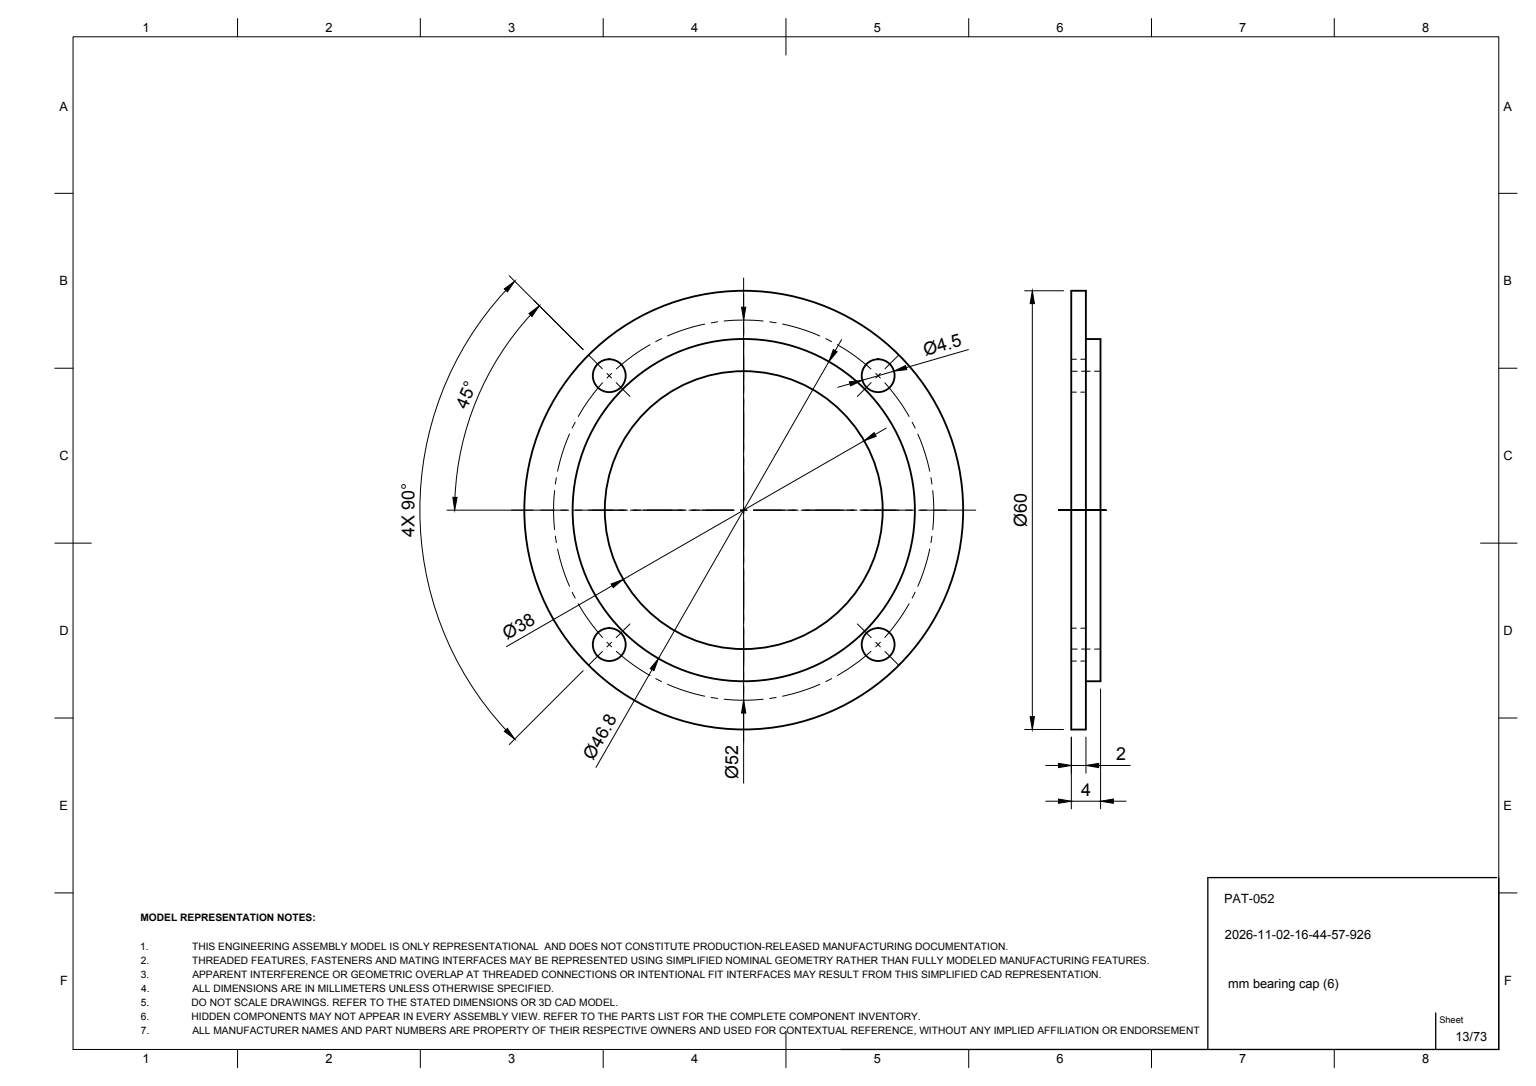
ISO-10303-21;
HEADER;
/* Generated by software containing ST-Developer
 * from STEP Tools, Inc. (www.steptools.com) 
 */

FILE_DESCRIPTION(
/* description */ ('Hand-crank gear train demonstrator'),
/* implementation_level */ '2;1');

FILE_NAME(
/* name */ 'mm bearing cap (6).step',
/* time_stamp */ '2026-10-28T03:22:13-07:00',
/* author */ (''),
/* organization */ (''),
/* preprocessor_version */ 'ST-DEVELOPER v20.2',
/* originating_system */ 'Autodesk Translation Framework v15.17.0.0',
/* authorisation */ '');

FILE_SCHEMA (('AUTOMOTIVE_DESIGN { 1 0 10303 214 3 1 1 }'));
ENDSEC;

DATA;
#10=MECHANICAL_DESIGN_GEOMETRIC_PRESENTATION_REPRESENTATION('',(#1198),#62758);
#1070=SHAPE_REPRESENTATION_RELATIONSHIP('SRR','None',#63042,#1134);
#1134=ADVANCED_BREP_SHAPE_REPRESENTATION('',(#1276),#62696);
#1198=STYLED_ITEM('',(#63462),#1276);
#1276=MANIFOLD_SOLID_BREP('Body1',#16379);
#1465=FACE_BOUND('',#3306,.T.);
#1466=FACE_BOUND('',#3310,.T.);
#1467=FACE_BOUND('',#3311,.T.);
#1468=FACE_BOUND('',#3312,.T.);
#1469=FACE_BOUND('',#3313,.T.);
#1470=FACE_BOUND('',#3314,.T.);
#1471=FACE_BOUND('',#3316,.T.);
#1472=FACE_BOUND('',#3317,.T.);
#1473=FACE_BOUND('',#3318,.T.);
#1474=FACE_BOUND('',#3319,.T.);
#1475=FACE_BOUND('',#3320,.T.);
#1676=PLANE('',#17450);
#1677=PLANE('',#17457);
#1678=PLANE('',#17458);
#2241=FACE_OUTER_BOUND('',#3300,.T.);
#2242=FACE_OUTER_BOUND('',#3301,.T.);
#2243=FACE_OUTER_BOUND('',#3302,.T.);
#2244=FACE_OUTER_BOUND('',#3303,.T.);
#2245=FACE_OUTER_BOUND('',#3304,.T.);
#2246=FACE_OUTER_BOUND('',#3305,.T.);
#2247=FACE_OUTER_BOUND('',#3307,.T.);
#2248=FACE_OUTER_BOUND('',#3308,.T.);
#2249=FACE_OUTER_BOUND('',#3309,.T.);
#2250=FACE_OUTER_BOUND('',#3315,.T.);
#3300=EDGE_LOOP('',(#11375,#11376,#11377,#11378));
#3301=EDGE_LOOP('',(#11379,#11380,#11381,#11382));
#3302=EDGE_LOOP('',(#11383,#11384,#11385,#11386));
#3303=EDGE_LOOP('',(#11387,#11388,#11389,#11390));
#3304=EDGE_LOOP('',(#11391,#11392,#11393,#11394));
#3305=EDGE_LOOP('',(#11395));
#3306=EDGE_LOOP('',(#11396));
#3307=EDGE_LOOP('',(#11397,#11398,#11399,#11400));
#3308=EDGE_LOOP('',(#11401,#11402,#11403,#11404));
#3309=EDGE_LOOP('',(#11405));
#3310=EDGE_LOOP('',(#11406));
#3311=EDGE_LOOP('',(#11407));
#3312=EDGE_LOOP('',(#11408));
#3313=EDGE_LOOP('',(#11409));
#3314=EDGE_LOOP('',(#11410));
#3315=EDGE_LOOP('',(#11411));
#3316=EDGE_LOOP('',(#11412));
#3317=EDGE_LOOP('',(#11413));
#3318=EDGE_LOOP('',(#11414));
#3319=EDGE_LOOP('',(#11415));
#3320=EDGE_LOOP('',(#11416));
#4409=LINE('',#23892,#5541);
#4410=LINE('',#23898,#5542);
#4411=LINE('',#23904,#5543);
#4412=LINE('',#23910,#5544);
#4413=LINE('',#23916,#5545);
#4414=LINE('',#23923,#5546);
#4415=LINE('',#23929,#5547);
#5541=VECTOR('',#19512,0.225000000000001);
#5542=VECTOR('',#19519,0.225000000000001);
#5543=VECTOR('',#19526,0.225000000000001);
#5544=VECTOR('',#19533,0.225000000000001);
#5545=VECTOR('',#19540,2.34);
#5546=VECTOR('',#19549,1.9);
#5547=VECTOR('',#19556,3.);
#6697=CIRCLE('',#17436,0.225000000000001);
#6698=CIRCLE('',#17437,0.225000000000001);
#6699=CIRCLE('',#17439,0.225000000000001);
#6700=CIRCLE('',#17440,0.225000000000001);
#6701=CIRCLE('',#17442,0.225000000000001);
#6702=CIRCLE('',#17443,0.225000000000001);
#6703=CIRCLE('',#17445,0.225000000000001);
#6704=CIRCLE('',#17446,0.225000000000001);
#6705=CIRCLE('',#17448,2.34);
#6706=CIRCLE('',#17449,2.34);
#6707=CIRCLE('',#17451,1.9);
#6708=CIRCLE('',#17453,1.9);
#6709=CIRCLE('',#17455,3.);
#6710=CIRCLE('',#17456,3.);
#7391=VERTEX_POINT('',#23889);
#7392=VERTEX_POINT('',#23891);
#7393=VERTEX_POINT('',#23895);
#7394=VERTEX_POINT('',#23897);
#7395=VERTEX_POINT('',#23901);
#7396=VERTEX_POINT('',#23903);
#7397=VERTEX_POINT('',#23907);
#7398=VERTEX_POINT('',#23909);
#7399=VERTEX_POINT('',#23913);
#7400=VERTEX_POINT('',#23915);
#7401=VERTEX_POINT('',#23919);
#7402=VERTEX_POINT('',#23922);
#7403=VERTEX_POINT('',#23926);
#7404=VERTEX_POINT('',#23928);
#8939=EDGE_CURVE('',#7391,#7391,#6697,.T.);
#8940=EDGE_CURVE('',#7391,#7392,#4409,.T.);
#8941=EDGE_CURVE('',#7392,#7392,#6698,.T.);
#8942=EDGE_CURVE('',#7393,#7393,#6699,.T.);
#8943=EDGE_CURVE('',#7393,#7394,#4410,.T.);
#8944=EDGE_CURVE('',#7394,#7394,#6700,.T.);
#8945=EDGE_CURVE('',#7395,#7395,#6701,.T.);
#8946=EDGE_CURVE('',#7395,#7396,#4411,.T.);
#8947=EDGE_CURVE('',#7396,#7396,#6702,.T.);
#8948=EDGE_CURVE('',#7397,#7397,#6703,.T.);
#8949=EDGE_CURVE('',#7397,#7398,#4412,.T.);
#8950=EDGE_CURVE('',#7398,#7398,#6704,.T.);
#8951=EDGE_CURVE('',#7399,#7399,#6705,.T.);
#8952=EDGE_CURVE('',#7399,#7400,#4413,.T.);
#8953=EDGE_CURVE('',#7400,#7400,#6706,.T.);
#8954=EDGE_CURVE('',#7401,#7401,#6707,.T.);
#8955=EDGE_CURVE('',#7401,#7402,#4414,.T.);
#8956=EDGE_CURVE('',#7402,#7402,#6708,.T.);
#8957=EDGE_CURVE('',#7403,#7403,#6709,.T.);
#8958=EDGE_CURVE('',#7403,#7404,#4415,.T.);
#8959=EDGE_CURVE('',#7404,#7404,#6710,.T.);
#11375=ORIENTED_EDGE('',*,*,#8939,.F.);
#11376=ORIENTED_EDGE('',*,*,#8940,.T.);
#11377=ORIENTED_EDGE('',*,*,#8941,.F.);
#11378=ORIENTED_EDGE('',*,*,#8940,.F.);
#11379=ORIENTED_EDGE('',*,*,#8942,.F.);
#11380=ORIENTED_EDGE('',*,*,#8943,.T.);
#11381=ORIENTED_EDGE('',*,*,#8944,.F.);
#11382=ORIENTED_EDGE('',*,*,#8943,.F.);
#11383=ORIENTED_EDGE('',*,*,#8945,.F.);
#11384=ORIENTED_EDGE('',*,*,#8946,.T.);
#11385=ORIENTED_EDGE('',*,*,#8947,.F.);
#11386=ORIENTED_EDGE('',*,*,#8946,.F.);
#11387=ORIENTED_EDGE('',*,*,#8948,.F.);
#11388=ORIENTED_EDGE('',*,*,#8949,.T.);
#11389=ORIENTED_EDGE('',*,*,#8950,.F.);
#11390=ORIENTED_EDGE('',*,*,#8949,.F.);
#11391=ORIENTED_EDGE('',*,*,#8951,.F.);
#11392=ORIENTED_EDGE('',*,*,#8952,.T.);
#11393=ORIENTED_EDGE('',*,*,#8953,.F.);
#11394=ORIENTED_EDGE('',*,*,#8952,.F.);
#11395=ORIENTED_EDGE('',*,*,#8951,.T.);
#11396=ORIENTED_EDGE('',*,*,#8954,.T.);
#11397=ORIENTED_EDGE('',*,*,#8954,.F.);
#11398=ORIENTED_EDGE('',*,*,#8955,.T.);
#11399=ORIENTED_EDGE('',*,*,#8956,.T.);
#11400=ORIENTED_EDGE('',*,*,#8955,.F.);
#11401=ORIENTED_EDGE('',*,*,#8957,.F.);
#11402=ORIENTED_EDGE('',*,*,#8958,.T.);
#11403=ORIENTED_EDGE('',*,*,#8959,.T.);
#11404=ORIENTED_EDGE('',*,*,#8958,.F.);
#11405=ORIENTED_EDGE('',*,*,#8957,.T.);
#11406=ORIENTED_EDGE('',*,*,#8953,.T.);
#11407=ORIENTED_EDGE('',*,*,#8950,.T.);
#11408=ORIENTED_EDGE('',*,*,#8947,.T.);
#11409=ORIENTED_EDGE('',*,*,#8944,.T.);
#11410=ORIENTED_EDGE('',*,*,#8941,.T.);
#11411=ORIENTED_EDGE('',*,*,#8959,.F.);
#11412=ORIENTED_EDGE('',*,*,#8956,.F.);
#11413=ORIENTED_EDGE('',*,*,#8948,.T.);
#11414=ORIENTED_EDGE('',*,*,#8945,.T.);
#11415=ORIENTED_EDGE('',*,*,#8942,.T.);
#11416=ORIENTED_EDGE('',*,*,#8939,.T.);
#15239=CYLINDRICAL_SURFACE('',#17435,0.225000000000001);
#15240=CYLINDRICAL_SURFACE('',#17438,0.225000000000001);
#15241=CYLINDRICAL_SURFACE('',#17441,0.225000000000001);
#15242=CYLINDRICAL_SURFACE('',#17444,0.225000000000001);
#15243=CYLINDRICAL_SURFACE('',#17447,2.34);
#15244=CYLINDRICAL_SURFACE('',#17452,1.9);
#15245=CYLINDRICAL_SURFACE('',#17454,3.);
#15551=ADVANCED_FACE('',(#2241),#15239,.F.);
#15552=ADVANCED_FACE('',(#2242),#15240,.F.);
#15553=ADVANCED_FACE('',(#2243),#15241,.F.);
#15554=ADVANCED_FACE('',(#2244),#15242,.F.);
#15555=ADVANCED_FACE('',(#2245),#15243,.T.);
#15556=ADVANCED_FACE('',(#2246,#1465),#1676,.T.);
#15557=ADVANCED_FACE('',(#2247),#15244,.F.);
#15558=ADVANCED_FACE('',(#2248),#15245,.T.);
#15559=ADVANCED_FACE('',(#2249,#1466,#1467,#1468,#1469,#1470),#1677,.T.);
#15560=ADVANCED_FACE('',(#2250,#1471,#1472,#1473,#1474,#1475),#1678,.F.);
#16379=CLOSED_SHELL('',(#15551,#15552,#15553,#15554,#15555,#15556,#15557,
#15558,#15559,#15560));
#17434=AXIS2_PLACEMENT_3D('',#23887,#19506,#19507);
#17435=AXIS2_PLACEMENT_3D('',#23888,#19508,#19509);
#17436=AXIS2_PLACEMENT_3D('',#23890,#19510,#19511);
#17437=AXIS2_PLACEMENT_3D('',#23893,#19513,#19514);
#17438=AXIS2_PLACEMENT_3D('',#23894,#19515,#19516);
#17439=AXIS2_PLACEMENT_3D('',#23896,#19517,#19518);
#17440=AXIS2_PLACEMENT_3D('',#23899,#19520,#19521);
#17441=AXIS2_PLACEMENT_3D('',#23900,#19522,#19523);
#17442=AXIS2_PLACEMENT_3D('',#23902,#19524,#19525);
#17443=AXIS2_PLACEMENT_3D('',#23905,#19527,#19528);
#17444=AXIS2_PLACEMENT_3D('',#23906,#19529,#19530);
#17445=AXIS2_PLACEMENT_3D('',#23908,#19531,#19532);
#17446=AXIS2_PLACEMENT_3D('',#23911,#19534,#19535);
#17447=AXIS2_PLACEMENT_3D('',#23912,#19536,#19537);
#17448=AXIS2_PLACEMENT_3D('',#23914,#19538,#19539);
#17449=AXIS2_PLACEMENT_3D('',#23917,#19541,#19542);
#17450=AXIS2_PLACEMENT_3D('',#23918,#19543,#19544);
#17451=AXIS2_PLACEMENT_3D('',#23920,#19545,#19546);
#17452=AXIS2_PLACEMENT_3D('',#23921,#19547,#19548);
#17453=AXIS2_PLACEMENT_3D('',#23924,#19550,#19551);
#17454=AXIS2_PLACEMENT_3D('',#23925,#19552,#19553);
#17455=AXIS2_PLACEMENT_3D('',#23927,#19554,#19555);
#17456=AXIS2_PLACEMENT_3D('',#23930,#19557,#19558);
#17457=AXIS2_PLACEMENT_3D('',#23931,#19559,#19560);
#17458=AXIS2_PLACEMENT_3D('',#23932,#19561,#19562);
#19506=DIRECTION('axis',(0.,0.,1.));
#19507=DIRECTION('refdir',(1.,0.,0.));
#19508=DIRECTION('center_axis',(0.,1.,0.));
#19509=DIRECTION('ref_axis',(1.,0.,0.));
#19510=DIRECTION('center_axis',(0.,1.,0.));
#19511=DIRECTION('ref_axis',(1.,0.,0.));
#19512=DIRECTION('',(0.,1.,0.));
#19513=DIRECTION('center_axis',(0.,-1.,0.));
#19514=DIRECTION('ref_axis',(1.,0.,0.));
#19515=DIRECTION('center_axis',(0.,1.,0.));
#19516=DIRECTION('ref_axis',(1.,0.,0.));
#19517=DIRECTION('center_axis',(0.,1.,0.));
#19518=DIRECTION('ref_axis',(1.,0.,0.));
#19519=DIRECTION('',(0.,1.,0.));
#19520=DIRECTION('center_axis',(0.,-1.,0.));
#19521=DIRECTION('ref_axis',(1.,0.,0.));
#19522=DIRECTION('center_axis',(0.,1.,0.));
#19523=DIRECTION('ref_axis',(1.,0.,0.));
#19524=DIRECTION('center_axis',(0.,1.,0.));
#19525=DIRECTION('ref_axis',(1.,0.,0.));
#19526=DIRECTION('',(0.,1.,0.));
#19527=DIRECTION('center_axis',(0.,-1.,0.));
#19528=DIRECTION('ref_axis',(1.,0.,0.));
#19529=DIRECTION('center_axis',(0.,1.,0.));
#19530=DIRECTION('ref_axis',(1.,0.,0.));
#19531=DIRECTION('center_axis',(0.,1.,0.));
#19532=DIRECTION('ref_axis',(1.,0.,0.));
#19533=DIRECTION('',(0.,1.,0.));
#19534=DIRECTION('center_axis',(0.,-1.,0.));
#19535=DIRECTION('ref_axis',(1.,0.,0.));
#19536=DIRECTION('center_axis',(0.,1.,0.));
#19537=DIRECTION('ref_axis',(1.,0.,0.));
#19538=DIRECTION('center_axis',(0.,1.,0.));
#19539=DIRECTION('ref_axis',(1.,0.,0.));
#19540=DIRECTION('',(0.,-1.,0.));
#19541=DIRECTION('center_axis',(0.,-1.,0.));
#19542=DIRECTION('ref_axis',(1.,0.,0.));
#19543=DIRECTION('center_axis',(0.,1.,0.));
#19544=DIRECTION('ref_axis',(1.,0.,0.));
#19545=DIRECTION('center_axis',(0.,-1.,0.));
#19546=DIRECTION('ref_axis',(1.,0.,0.));
#19547=DIRECTION('center_axis',(0.,1.,0.));
#19548=DIRECTION('ref_axis',(1.,0.,0.));
#19549=DIRECTION('',(0.,-1.,0.));
#19550=DIRECTION('center_axis',(0.,-1.,0.));
#19551=DIRECTION('ref_axis',(1.,0.,0.));
#19552=DIRECTION('center_axis',(0.,1.,0.));
#19553=DIRECTION('ref_axis',(1.,0.,0.));
#19554=DIRECTION('center_axis',(0.,1.,0.));
#19555=DIRECTION('ref_axis',(1.,0.,0.));
#19556=DIRECTION('',(0.,-1.,0.));
#19557=DIRECTION('center_axis',(0.,1.,0.));
#19558=DIRECTION('ref_axis',(1.,0.,0.));
#19559=DIRECTION('center_axis',(0.,1.,0.));
#19560=DIRECTION('ref_axis',(1.,0.,0.));
#19561=DIRECTION('center_axis',(0.,1.,0.));
#19562=DIRECTION('ref_axis',(1.,0.,0.));
#23887=CARTESIAN_POINT('',(0.,0.,0.));
#23888=CARTESIAN_POINT('Origin',(16.161522368915,-2.7,7.16152236891498));
#23889=CARTESIAN_POINT('',(15.936522368915,-2.6,7.16152236891498));
#23890=CARTESIAN_POINT('Origin',(16.161522368915,-2.6,7.16152236891498));
#23891=CARTESIAN_POINT('',(15.936522368915,-2.4,7.16152236891498));
#23892=CARTESIAN_POINT('',(15.936522368915,-2.7,7.16152236891498));
#23893=CARTESIAN_POINT('Origin',(16.161522368915,-2.4,7.16152236891498));
#23894=CARTESIAN_POINT('Origin',(16.161522368915,-2.7,10.838477631085));
#23895=CARTESIAN_POINT('',(15.936522368915,-2.6,10.838477631085));
#23896=CARTESIAN_POINT('Origin',(16.161522368915,-2.6,10.838477631085));
#23897=CARTESIAN_POINT('',(15.936522368915,-2.4,10.838477631085));
#23898=CARTESIAN_POINT('',(15.936522368915,-2.7,10.838477631085));
#23899=CARTESIAN_POINT('Origin',(16.161522368915,-2.4,10.838477631085));
#23900=CARTESIAN_POINT('Origin',(19.838477631085,-2.7,10.838477631085));
#23901=CARTESIAN_POINT('',(19.613477631085,-2.6,10.838477631085));
#23902=CARTESIAN_POINT('Origin',(19.838477631085,-2.6,10.838477631085));
#23903=CARTESIAN_POINT('',(19.613477631085,-2.4,10.838477631085));
#23904=CARTESIAN_POINT('',(19.613477631085,-2.7,10.838477631085));
#23905=CARTESIAN_POINT('Origin',(19.838477631085,-2.4,10.838477631085));
#23906=CARTESIAN_POINT('Origin',(19.838477631085,-2.7,7.16152236891498));
#23907=CARTESIAN_POINT('',(19.613477631085,-2.6,7.16152236891498));
#23908=CARTESIAN_POINT('Origin',(19.838477631085,-2.6,7.16152236891498));
#23909=CARTESIAN_POINT('',(19.613477631085,-2.4,7.16152236891498));
#23910=CARTESIAN_POINT('',(19.613477631085,-2.7,7.16152236891498));
#23911=CARTESIAN_POINT('Origin',(19.838477631085,-2.4,7.16152236891498));
#23912=CARTESIAN_POINT('Origin',(18.,-2.4,9.));
#23913=CARTESIAN_POINT('',(15.66,-2.2,9.));
#23914=CARTESIAN_POINT('Origin',(18.,-2.2,9.));
#23915=CARTESIAN_POINT('',(15.66,-2.4,9.));
#23916=CARTESIAN_POINT('',(15.66,-2.4,9.));
#23917=CARTESIAN_POINT('Origin',(18.,-2.4,9.));
#23918=CARTESIAN_POINT('Origin',(18.,-2.2,9.));
#23919=CARTESIAN_POINT('',(16.1,-2.2,9.));
#23920=CARTESIAN_POINT('Origin',(18.,-2.2,9.));
#23921=CARTESIAN_POINT('Origin',(18.,-2.6,9.));
#23922=CARTESIAN_POINT('',(16.1,-2.6,9.));
#23923=CARTESIAN_POINT('',(16.1,-2.6,9.));
#23924=CARTESIAN_POINT('Origin',(18.,-2.6,9.));
#23925=CARTESIAN_POINT('Origin',(18.,-2.6,9.));
#23926=CARTESIAN_POINT('',(15.,-2.4,9.));
#23927=CARTESIAN_POINT('Origin',(18.,-2.4,9.));
#23928=CARTESIAN_POINT('',(15.,-2.6,9.));
#23929=CARTESIAN_POINT('',(15.,-2.6,9.));
#23930=CARTESIAN_POINT('Origin',(18.,-2.6,9.));
#23931=CARTESIAN_POINT('Origin',(18.,-2.4,9.));
#23932=CARTESIAN_POINT('Origin',(18.,-2.6,9.));
#62622=UNCERTAINTY_MEASURE_WITH_UNIT(LENGTH_MEASURE(0.001),#62759,
'DISTANCE_ACCURACY_VALUE',
'Maximum model space distance between geometric entities at asserted c
onnectivities');
#62684=UNCERTAINTY_MEASURE_WITH_UNIT(LENGTH_MEASURE(0.001),#62759,
'DISTANCE_ACCURACY_VALUE',
'Maximum model space distance between geometric entities at asserted c
onnectivities');
#62696=(
GEOMETRIC_REPRESENTATION_CONTEXT(3)
GLOBAL_UNCERTAINTY_ASSIGNED_CONTEXT((#62622))
GLOBAL_UNIT_ASSIGNED_CONTEXT((#62759,#62761,#62762))
REPRESENTATION_CONTEXT('','3D')
);
#62758=(
GEOMETRIC_REPRESENTATION_CONTEXT(3)
GLOBAL_UNCERTAINTY_ASSIGNED_CONTEXT((#62684))
GLOBAL_UNIT_ASSIGNED_CONTEXT((#62759,#62761,#62762))
REPRESENTATION_CONTEXT('','3D')
);
#62759=(
LENGTH_UNIT()
NAMED_UNIT(*)
SI_UNIT(.CENTI.,.METRE.)
);
#62761=(
NAMED_UNIT(*)
PLANE_ANGLE_UNIT()
SI_UNIT($,.RADIAN.)
);
#62762=(
NAMED_UNIT(*)
SI_UNIT($,.STERADIAN.)
SOLID_ANGLE_UNIT()
);
#62774=SHAPE_DEFINITION_REPRESENTATION(#62847,#63042);
#62847=PRODUCT_DEFINITION_SHAPE('',$,#63116);
#63042=SHAPE_REPRESENTATION('',(#17434),#62696);
#63104=PRODUCT_DEFINITION_CONTEXT('part definition',#63325,'design');
#63116=PRODUCT_DEFINITION('mm bearing cap (6)','mm bearing cap (6)',#63189,
#63104);
#63189=PRODUCT_DEFINITION_FORMATION('',$,#63338);
#63325=APPLICATION_CONTEXT(
'Core Data for Automotive Mechanical Design Process');
#63326=PRODUCT_CONTEXT('part definition',#63325,'mechanical');
#63338=PRODUCT('mm bearing cap (6)','mm bearing cap (6)','mm bearing cap (6)',
(#63326));
#63456=COLOUR_RGB('Grey',0.48,0.52,0.57);
#63457=FILL_AREA_STYLE_COLOUR('',#63456);
#63458=FILL_AREA_STYLE('',(#63457));
#63459=SURFACE_STYLE_FILL_AREA(#63458);
#63460=SURFACE_SIDE_STYLE('',(#63459));
#63461=SURFACE_STYLE_USAGE(.BOTH.,#63460);
#63462=PRESENTATION_STYLE_ASSIGNMENT((#63461));
ENDSEC;
END-ISO-10303-21;
